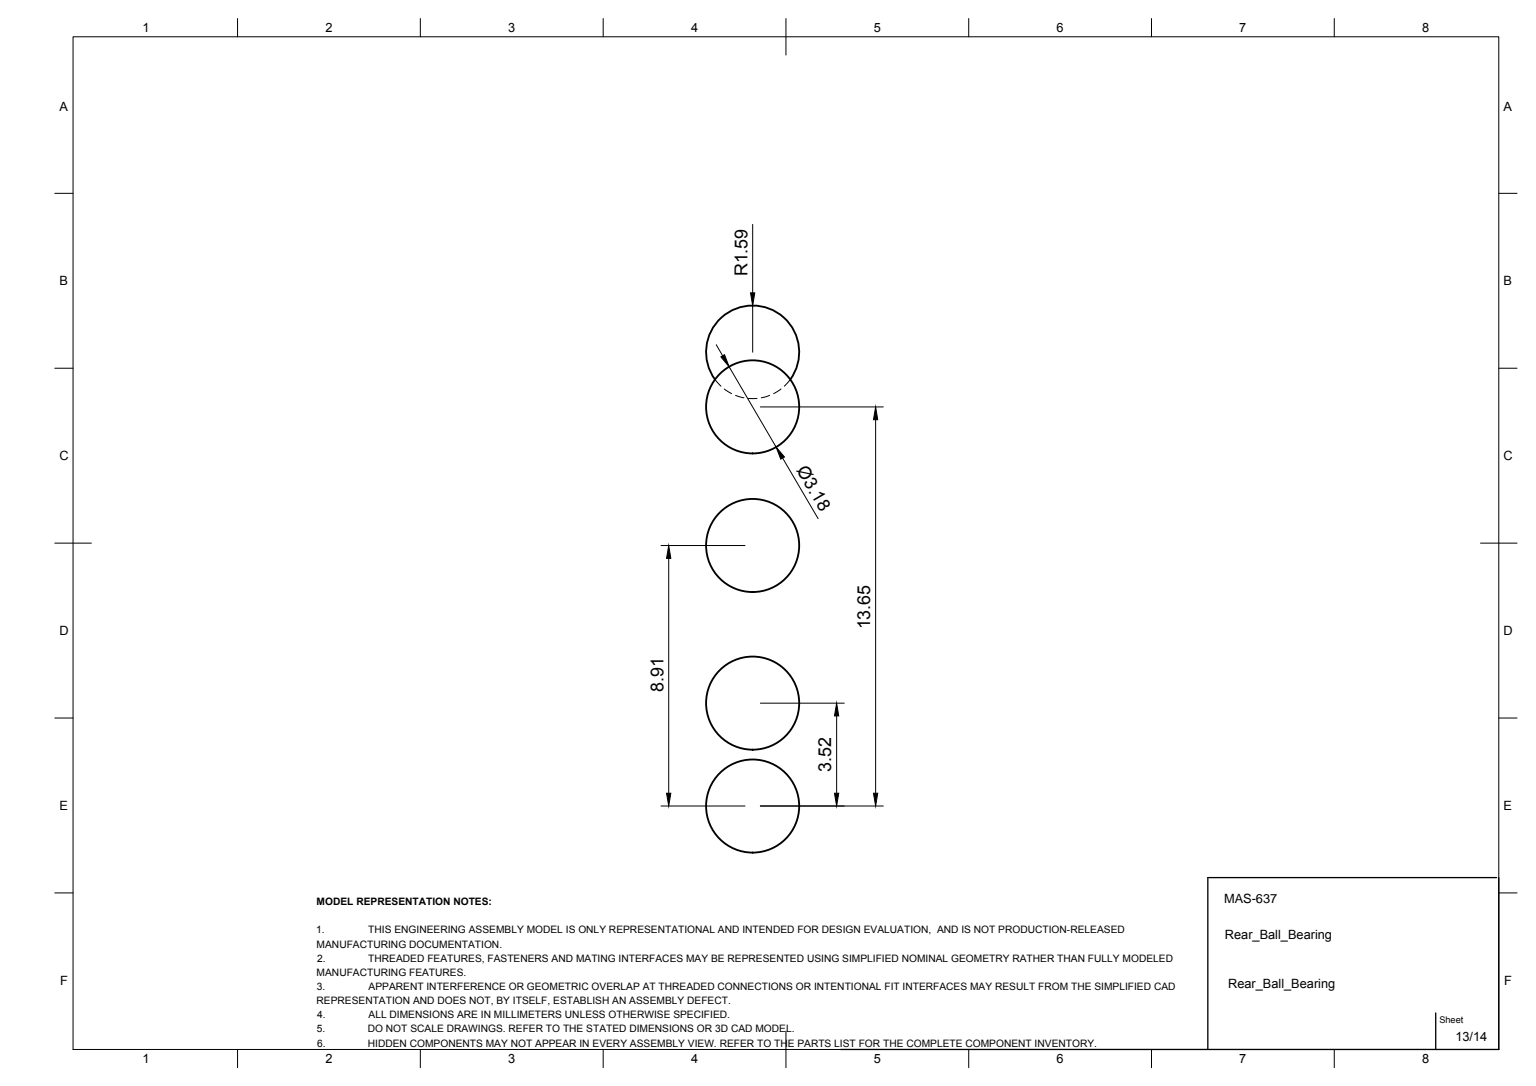
ISO-10303-21;
HEADER;
FILE_DESCRIPTION((''),'2;1');
FILE_NAME('Rear_Ball_Bearing.step','2026-10-09T10:11:57-07:00',(''),(''),'','','');
FILE_SCHEMA (('AUTOMOTIVE_DESIGN { 1 0 10303 214 3 1 1 }'));
ENDSEC;
DATA;
#10=MECHANICAL_DESIGN_GEOMETRIC_PRESENTATION_REPRESENTATION('',(#145,#146,#147,#148,#149,#150,#151,#152,#153),#13510);
#84=SPHERICAL_SURFACE('',#8500,1.59) ;
#85=SPHERICAL_SURFACE('',#8502,1.59) ;
#86=SPHERICAL_SURFACE('',#8504,1.59) ;
#87=SPHERICAL_SURFACE('',#8506,1.59) ;
#88=SPHERICAL_SURFACE('',#8508,1.59) ;
#89=SPHERICAL_SURFACE('',#8510,1.59) ;
#90=SPHERICAL_SURFACE('',#8512,1.59) ;
#91=SPHERICAL_SURFACE('',#8514,1.59) ;
#92=SPHERICAL_SURFACE('',#8516,1.59) ;
#106=SHAPE_REPRESENTATION_RELATIONSHIP('SRR','None',#13576,#121) ;
#121=ADVANCED_BREP_SHAPE_REPRESENTATION('',(#177,#178,#179,#180,#181,#182,
#183,#184,#185),#13508) ;
#145=STYLED_ITEM('',(#13650),#177) ;
#146=STYLED_ITEM('',(#13650),#178) ;
#147=STYLED_ITEM('',(#13650),#179) ;
#148=STYLED_ITEM('',(#13650),#180) ;
#149=STYLED_ITEM('',(#13650),#181) ;
#150=STYLED_ITEM('',(#13650),#182) ;
#151=STYLED_ITEM('',(#13650),#183) ;
#152=STYLED_ITEM('',(#13650),#184) ;
#153=STYLED_ITEM('',(#13650),#185) ;
#177=MANIFOLD_SOLID_BREP('Body1',#7394) ;
#178=MANIFOLD_SOLID_BREP('Body2',#7395) ;
#179=MANIFOLD_SOLID_BREP('Body3',#7396) ;
#180=MANIFOLD_SOLID_BREP('Body4',#7397) ;
#181=MANIFOLD_SOLID_BREP('Body5',#7398) ;
#182=MANIFOLD_SOLID_BREP('Body6',#7399) ;
#183=MANIFOLD_SOLID_BREP('Body7',#7400) ;
#184=MANIFOLD_SOLID_BREP('Body8',#7401) ;
#185=MANIFOLD_SOLID_BREP('Body9',#7402) ;
#1099=FACE_OUTER_BOUND('',#1624,.T.) ;
#1100=FACE_OUTER_BOUND('',#1625,.T.) ;
#1101=FACE_OUTER_BOUND('',#1626,.T.) ;
#1102=FACE_OUTER_BOUND('',#1627,.T.) ;
#1103=FACE_OUTER_BOUND('',#1628,.T.) ;
#1104=FACE_OUTER_BOUND('',#1629,.T.) ;
#1105=FACE_OUTER_BOUND('',#1630,.T.) ;
#1106=FACE_OUTER_BOUND('',#1631,.T.) ;
#1107=FACE_OUTER_BOUND('',#1632,.T.) ;
#1624=EDGE_LOOP('',(#6800,#6801)) ;
#1625=EDGE_LOOP('',(#6802,#6803)) ;
#1626=EDGE_LOOP('',(#6804,#6805)) ;
#1627=EDGE_LOOP('',(#6806,#6807)) ;
#1628=EDGE_LOOP('',(#6808,#6809)) ;
#1629=EDGE_LOOP('',(#6810,#6811)) ;
#1630=EDGE_LOOP('',(#6812,#6813)) ;
#1631=EDGE_LOOP('',(#6814,#6815)) ;
#1632=EDGE_LOOP('',(#6816,#6817)) ;
#3115=CIRCLE('',#8501,1.59) ;
#3116=CIRCLE('',#8503,1.59) ;
#3117=CIRCLE('',#8505,1.59) ;
#3118=CIRCLE('',#8507,1.58999999999999) ;
#3119=CIRCLE('',#8509,1.59) ;
#3120=CIRCLE('',#8511,1.59) ;
#3121=CIRCLE('',#8513,1.58999999999999) ;
#3122=CIRCLE('',#8515,1.59) ;
#3123=CIRCLE('',#8517,1.59) ;
#3766=VERTEX_POINT('',#13372) ;
#3767=VERTEX_POINT('',#13373) ;
#3768=VERTEX_POINT('',#13376) ;
#3769=VERTEX_POINT('',#13377) ;
#3770=VERTEX_POINT('',#13380) ;
#3771=VERTEX_POINT('',#13381) ;
#3772=VERTEX_POINT('',#13384) ;
#3773=VERTEX_POINT('',#13385) ;
#3774=VERTEX_POINT('',#13388) ;
#3775=VERTEX_POINT('',#13389) ;
#3776=VERTEX_POINT('',#13392) ;
#3777=VERTEX_POINT('',#13393) ;
#3778=VERTEX_POINT('',#13396) ;
#3779=VERTEX_POINT('',#13397) ;
#3780=VERTEX_POINT('',#13400) ;
#3781=VERTEX_POINT('',#13401) ;
#3782=VERTEX_POINT('',#13404) ;
#3783=VERTEX_POINT('',#13405) ;
#4787=EDGE_CURVE('',#3766,#3767,#3115,.T.) ;
#4788=EDGE_CURVE('',#3768,#3769,#3116,.T.) ;
#4789=EDGE_CURVE('',#3770,#3771,#3117,.T.) ;
#4790=EDGE_CURVE('',#3772,#3773,#3118,.T.) ;
#4791=EDGE_CURVE('',#3774,#3775,#3119,.T.) ;
#4792=EDGE_CURVE('',#3776,#3777,#3120,.T.) ;
#4793=EDGE_CURVE('',#3778,#3779,#3121,.T.) ;
#4794=EDGE_CURVE('',#3780,#3781,#3122,.T.) ;
#4795=EDGE_CURVE('',#3782,#3783,#3123,.T.) ;
#6800=ORIENTED_EDGE('',*,*,#4787,.T.) ;
#6801=ORIENTED_EDGE('',*,*,#4787,.F.) ;
#6802=ORIENTED_EDGE('',*,*,#4788,.T.) ;
#6803=ORIENTED_EDGE('',*,*,#4788,.F.) ;
#6804=ORIENTED_EDGE('',*,*,#4789,.T.) ;
#6805=ORIENTED_EDGE('',*,*,#4789,.F.) ;
#6806=ORIENTED_EDGE('',*,*,#4790,.T.) ;
#6807=ORIENTED_EDGE('',*,*,#4790,.F.) ;
#6808=ORIENTED_EDGE('',*,*,#4791,.T.) ;
#6809=ORIENTED_EDGE('',*,*,#4791,.F.) ;
#6810=ORIENTED_EDGE('',*,*,#4792,.T.) ;
#6811=ORIENTED_EDGE('',*,*,#4792,.F.) ;
#6812=ORIENTED_EDGE('',*,*,#4793,.T.) ;
#6813=ORIENTED_EDGE('',*,*,#4793,.F.) ;
#6814=ORIENTED_EDGE('',*,*,#4794,.T.) ;
#6815=ORIENTED_EDGE('',*,*,#4794,.F.) ;
#6816=ORIENTED_EDGE('',*,*,#4795,.T.) ;
#6817=ORIENTED_EDGE('',*,*,#4795,.F.) ;
#7349=ADVANCED_FACE('',(#1099),#84,.T.) ;
#7350=ADVANCED_FACE('',(#1100),#85,.T.) ;
#7351=ADVANCED_FACE('',(#1101),#86,.T.) ;
#7352=ADVANCED_FACE('',(#1102),#87,.T.) ;
#7353=ADVANCED_FACE('',(#1103),#88,.T.) ;
#7354=ADVANCED_FACE('',(#1104),#89,.T.) ;
#7355=ADVANCED_FACE('',(#1105),#90,.T.) ;
#7356=ADVANCED_FACE('',(#1106),#91,.T.) ;
#7357=ADVANCED_FACE('',(#1107),#92,.T.) ;
#7394=CLOSED_SHELL('',(#7349)) ;
#7395=CLOSED_SHELL('',(#7350)) ;
#7396=CLOSED_SHELL('',(#7351)) ;
#7397=CLOSED_SHELL('',(#7352)) ;
#7398=CLOSED_SHELL('',(#7353)) ;
#7399=CLOSED_SHELL('',(#7354)) ;
#7400=CLOSED_SHELL('',(#7355)) ;
#7401=CLOSED_SHELL('',(#7356)) ;
#7402=CLOSED_SHELL('',(#7357)) ;
#8499=AXIS2_PLACEMENT_3D('',#13370,#10912,#10913) ;
#8500=AXIS2_PLACEMENT_3D('',#13371,#10914,#10915) ;
#8501=AXIS2_PLACEMENT_3D('',#13374,#10916,#10917) ;
#8502=AXIS2_PLACEMENT_3D('',#13375,#10918,#10919) ;
#8503=AXIS2_PLACEMENT_3D('',#13378,#10920,#10921) ;
#8504=AXIS2_PLACEMENT_3D('',#13379,#10922,#10923) ;
#8505=AXIS2_PLACEMENT_3D('',#13382,#10924,#10925) ;
#8506=AXIS2_PLACEMENT_3D('',#13383,#10926,#10927) ;
#8507=AXIS2_PLACEMENT_3D('',#13386,#10928,#10929) ;
#8508=AXIS2_PLACEMENT_3D('',#13387,#10930,#10931) ;
#8509=AXIS2_PLACEMENT_3D('',#13390,#10932,#10933) ;
#8510=AXIS2_PLACEMENT_3D('',#13391,#10934,#10935) ;
#8511=AXIS2_PLACEMENT_3D('',#13394,#10936,#10937) ;
#8512=AXIS2_PLACEMENT_3D('',#13395,#10938,#10939) ;
#8513=AXIS2_PLACEMENT_3D('',#13398,#10940,#10941) ;
#8514=AXIS2_PLACEMENT_3D('',#13399,#10942,#10943) ;
#8515=AXIS2_PLACEMENT_3D('',#13402,#10944,#10945) ;
#8516=AXIS2_PLACEMENT_3D('',#13403,#10946,#10947) ;
#8517=AXIS2_PLACEMENT_3D('',#13406,#10948,#10949) ;
#10912=DIRECTION('axis',(0.,0.,1.)) ;
#10913=DIRECTION('refdir',(1.,0.,0.)) ;
#10914=DIRECTION('center_axis',(-1.,8.806904269217E-17,0.)) ;
#10915=DIRECTION('ref_axis',(0.,0.479425538604202,0.877582561890374)) ;
#10916=DIRECTION('center_axis',(-5.15252374060182E-17,-0.877582561890373,
0.479425538604203)) ;
#10917=DIRECTION('ref_axis',(0.,-0.479425538604203,-0.877582561890373)) ;
#10918=DIRECTION('center_axis',(-0.76604444311876,0.642787609686799,0.)) ;
#10919=DIRECTION('ref_axis',(0.308168795982251,0.367261269737027,0.877582561890331)) ;
#10920=DIRECTION('center_axis',(-0.564099197260303,-0.672267244914013,0.479425538604281)) ;
#10921=DIRECTION('ref_axis',(-0.308168795982252,-0.367261269737028,-0.87758256189033)) ;
#10922=DIRECTION('center_axis',(-0.173648177667033,0.98480775301219,0.)) ;
#10923=DIRECTION('ref_axis',(0.472141987409266,0.0832513711056207,0.877582561890483)) ;
#10924=DIRECTION('center_axis',(-0.864250110858048,-0.152390612624649,0.479425538604001)) ;
#10925=DIRECTION('ref_axis',(-0.472141987409265,-0.0832513711056204,-0.877582561890483)) ;
#10926=DIRECTION('center_axis',(0.50000000000019,0.866025403784329,0.)) ;
#10927=DIRECTION('ref_axis',(0.415194695654166,-0.239712769302159,0.87758256189041)) ;
#10928=DIRECTION('center_axis',(-0.760008792515227,0.438791280945371,0.479425538604137)) ;
#10929=DIRECTION('ref_axis',(-0.415194695654167,0.239712769302159,-0.877582561890409)) ;
#10930=DIRECTION('center_axis',(0.939692620785813,0.342020143325932,0.)) ;
#10931=DIRECTION('ref_axis',(0.16397319142762,-0.450512640842904,0.877582561890216)) ;
#10932=DIRECTION('center_axis',(-0.30015091359803,0.824657857538545,0.47942553860449)) ;
#10933=DIRECTION('ref_axis',(-0.16397319142762,0.450512640842903,-0.877582561890216)) ;
#10934=DIRECTION('center_axis',(0.939692620785813,-0.342020143325932,0.)) ;
#10935=DIRECTION('ref_axis',(-0.16397319142762,-0.450512640842904,0.877582561890216)) ;
#10936=DIRECTION('center_axis',(0.30015091359803,0.824657857538545,0.47942553860449)) ;
#10937=DIRECTION('ref_axis',(0.16397319142762,0.450512640842903,-0.877582561890216)) ;
#10938=DIRECTION('center_axis',(0.50000000000019,-0.866025403784329,0.)) ;
#10939=DIRECTION('ref_axis',(-0.415194695654166,-0.239712769302159,0.87758256189041)) ;
#10940=DIRECTION('center_axis',(0.760008792515227,0.438791280945371,0.479425538604137)) ;
#10941=DIRECTION('ref_axis',(0.415194695654167,0.239712769302159,-0.877582561890409)) ;
#10942=DIRECTION('center_axis',(-0.173648177667034,-0.98480775301219,0.)) ;
#10943=DIRECTION('ref_axis',(-0.472141987409265,0.0832513711056207,0.877582561890483)) ;
#10944=DIRECTION('center_axis',(0.864250110858048,-0.152390612624649,0.479425538604001)) ;
#10945=DIRECTION('ref_axis',(0.472141987409265,-0.0832513711056211,-0.877582561890483)) ;
#10946=DIRECTION('center_axis',(-0.76604444311876,-0.642787609686799,0.)) ;
#10947=DIRECTION('ref_axis',(-0.308168795982251,0.367261269737027,0.877582561890331)) ;
#10948=DIRECTION('center_axis',(0.564099197260303,-0.672267244914013,0.479425538604281)) ;
#10949=DIRECTION('ref_axis',(0.308168795982252,-0.367261269737028,-0.87758256189033)) ;
#13370=CARTESIAN_POINT('',(0.,0.,0.)) ;
#13371=CARTESIAN_POINT('Origin',(8.,0.,112.)) ;
#13372=CARTESIAN_POINT('',(6.41,2.52194706263551E-17,112.)) ;
#13373=CARTESIAN_POINT('',(9.59,-1.18572655880055E-16,112.)) ;
#13374=CARTESIAN_POINT('Origin',(8.,0.,112.)) ;
#13375=CARTESIAN_POINT('Origin',(6.12835554495,-5.14230087749,112.)) ;
#13376=CARTESIAN_POINT('',(4.91034488039118,-4.12026857808799,112.)) ;
#13377=CARTESIAN_POINT('',(7.34636620950883,-6.16433317689201,112.)) ;
#13378=CARTESIAN_POINT('Origin',(6.12835554495,-5.14230087749,112.)) ;
#13379=CARTESIAN_POINT('Origin',(1.38918542134,-7.8784620241,112.)) ;
#13380=CARTESIAN_POINT('',(1.11308481884942,-6.31261769681062,112.)) ;
#13381=CARTESIAN_POINT('',(1.66528602383058,-9.44430635138938,112.)) ;
#13382=CARTESIAN_POINT('Origin',(1.38918542134,-7.8784620241,112.)) ;
#13383=CARTESIAN_POINT('Origin',(-4.,-6.92820323028,112.)) ;
#13384=CARTESIAN_POINT('',(-3.2049999999997,-5.55122283826292,112.)) ;
#13385=CARTESIAN_POINT('',(-4.7950000000003,-8.30518362229708,112.)) ;
#13386=CARTESIAN_POINT('Origin',(-4.,-6.92820323028,112.)) ;
#13387=CARTESIAN_POINT('Origin',(-7.51754096629,-2.73616114661,112.)) ;
#13388=CARTESIAN_POINT('',(-6.02342969924056,-2.19234911872177,112.)) ;
#13389=CARTESIAN_POINT('',(-9.01165223333944,-3.27997317449823,112.)) ;
#13390=CARTESIAN_POINT('Origin',(-7.51754096629,-2.73616114661,112.)) ;
#13391=CARTESIAN_POINT('Origin',(-7.51754096629,2.73616114661,112.)) ;
#13392=CARTESIAN_POINT('',(-6.02342969924056,2.19234911872177,112.)) ;
#13393=CARTESIAN_POINT('',(-9.01165223333944,3.27997317449823,112.)) ;
#13394=CARTESIAN_POINT('Origin',(-7.51754096629,2.73616114661,112.)) ;
#13395=CARTESIAN_POINT('Origin',(-4.,6.92820323028,112.)) ;
#13396=CARTESIAN_POINT('',(-3.2049999999997,5.55122283826292,112.)) ;
#13397=CARTESIAN_POINT('',(-4.7950000000003,8.30518362229708,112.)) ;
#13398=CARTESIAN_POINT('Origin',(-4.,6.92820323028,112.)) ;
#13399=CARTESIAN_POINT('Origin',(1.38918542134,7.8784620241,112.)) ;
#13400=CARTESIAN_POINT('',(1.11308481884942,6.31261769681062,112.)) ;
#13401=CARTESIAN_POINT('',(1.66528602383058,9.44430635138938,112.)) ;
#13402=CARTESIAN_POINT('Origin',(1.38918542134,7.8784620241,112.)) ;
#13403=CARTESIAN_POINT('Origin',(6.12835554495,5.14230087749,112.)) ;
#13404=CARTESIAN_POINT('',(4.91034488039118,4.12026857808799,112.)) ;
#13405=CARTESIAN_POINT('',(7.34636620950883,6.16433317689201,112.)) ;
#13406=CARTESIAN_POINT('Origin',(6.12835554495,5.14230087749,112.)) ;
#13491=UNCERTAINTY_MEASURE_WITH_UNIT(LENGTH_MEASURE(0.01),#13511,
'DISTANCE_ACCURACY_VALUE',
'Maximum model space distance between geometric entities at asserted c
onnectivities') ;
#13493=UNCERTAINTY_MEASURE_WITH_UNIT(LENGTH_MEASURE(0.01),#13511,
'DISTANCE_ACCURACY_VALUE',
'Maximum model space distance between geometric entities at asserted c
onnectivities') ;
#13508=(
GEOMETRIC_REPRESENTATION_CONTEXT(3)
GLOBAL_UNCERTAINTY_ASSIGNED_CONTEXT((#13491))
GLOBAL_UNIT_ASSIGNED_CONTEXT((#13511,#13513,#13514))
REPRESENTATION_CONTEXT('','3D')
) ;
#13510=(
GEOMETRIC_REPRESENTATION_CONTEXT(3)
GLOBAL_UNCERTAINTY_ASSIGNED_CONTEXT((#13493))
GLOBAL_UNIT_ASSIGNED_CONTEXT((#13511,#13513,#13514))
REPRESENTATION_CONTEXT('','3D')
) ;
#13511=(
LENGTH_UNIT()
NAMED_UNIT(*)
SI_UNIT(.MILLI.,.METRE.)
) ;
#13513=(
NAMED_UNIT(*)
PLANE_ANGLE_UNIT()
SI_UNIT($,.RADIAN.)
) ;
#13514=(
NAMED_UNIT(*)
SI_UNIT($,.STERADIAN.)
SOLID_ANGLE_UNIT()
) ;
#13529=SHAPE_DEFINITION_REPRESENTATION(#13545,#13576) ;
#13545=PRODUCT_DEFINITION_SHAPE('',$,#13593) ;
#13576=SHAPE_REPRESENTATION('',(#8499),#13508) ;
#13578=PRODUCT_DEFINITION_CONTEXT('part definition',#13628,'design') ;
#13593=PRODUCT_DEFINITION('Rear_Ball_Bearing','Rear_Ball_Bearing',#13609,
#13578) ;
#13609=PRODUCT_DEFINITION_FORMATION('',$,#13644) ;
#13628=APPLICATION_CONTEXT(
'Core Data for Automotive Mechanical Design Process') ;
#13629=PRODUCT_CONTEXT('part definition',#13628,'mechanical') ;
#13644=PRODUCT('Rear_Ball_Bearing','Rear_Ball_Bearing',$,(#13629)) ;
#13650=PRESENTATION_STYLE_ASSIGNMENT((#13655)) ;
#13655=SURFACE_STYLE_USAGE(.BOTH.,#13660) ;
#13660=SURFACE_SIDE_STYLE('',(#13665)) ;
#13665=SURFACE_STYLE_FILL_AREA(#13670) ;
#13670=FILL_AREA_STYLE('Opaque(144,144,144)',(#13675)) ;
#13675=FILL_AREA_STYLE_COLOUR('Opaque(144,144,144)',#13680) ;
#13680=COLOUR_RGB('Opaque(144,144,144)', 0.40784314, 0.44705882, 0.49803922) ;
ENDSEC;
END-ISO-10303-21;
